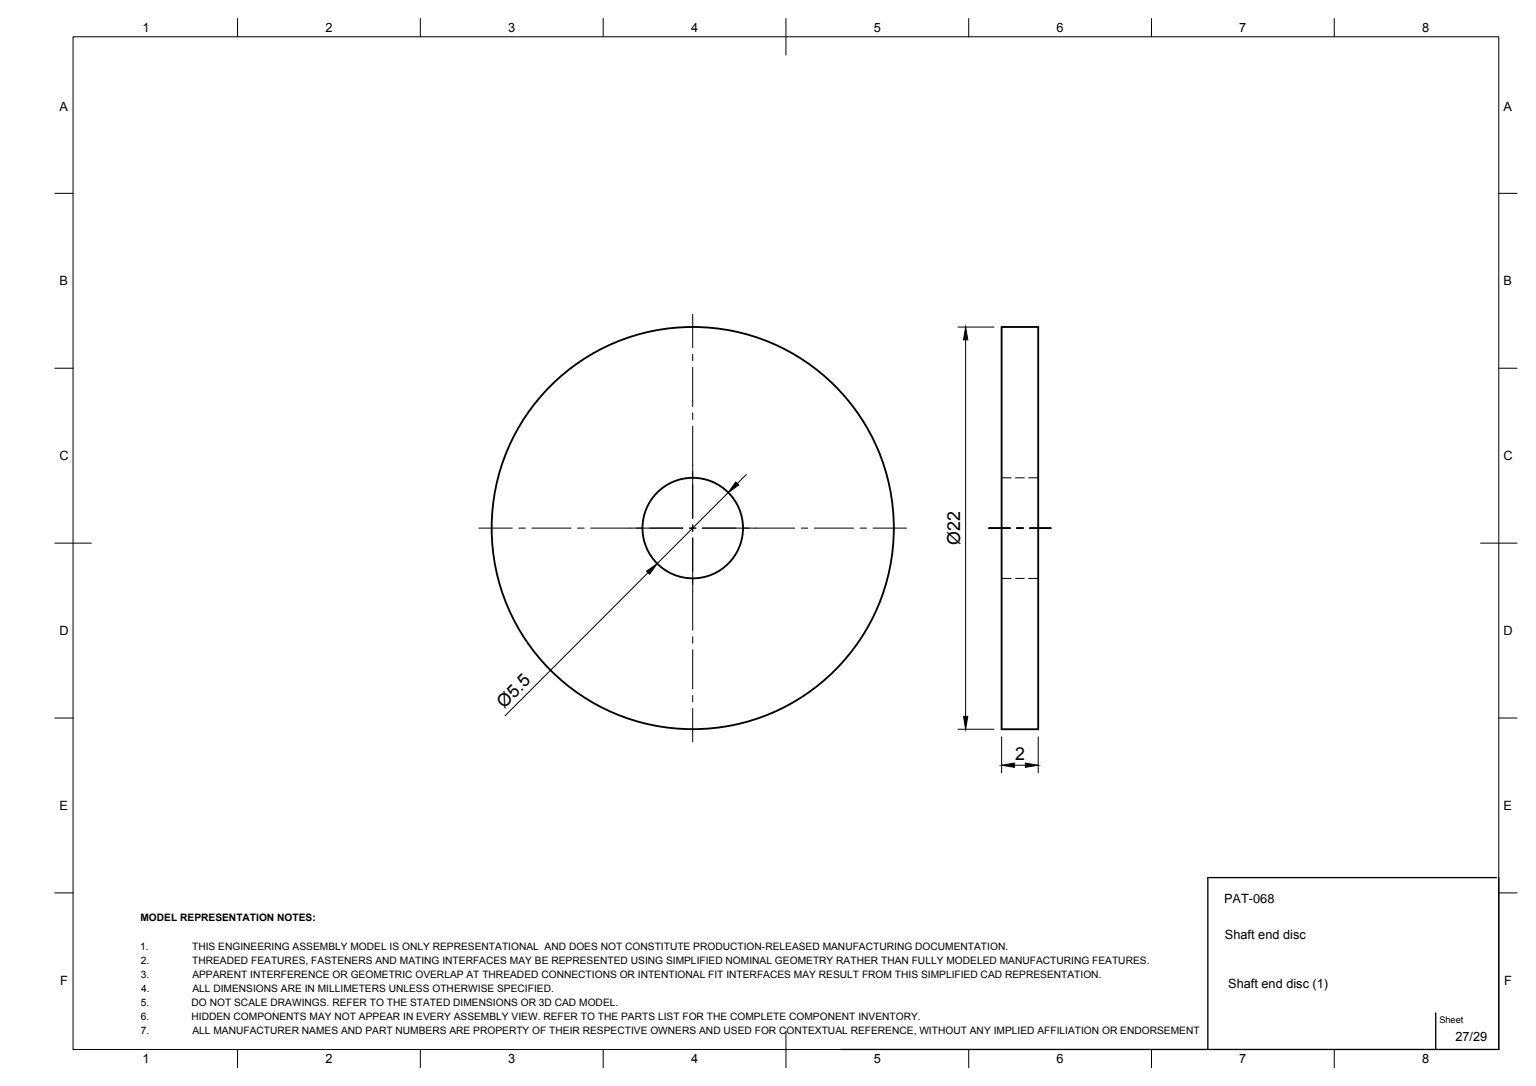
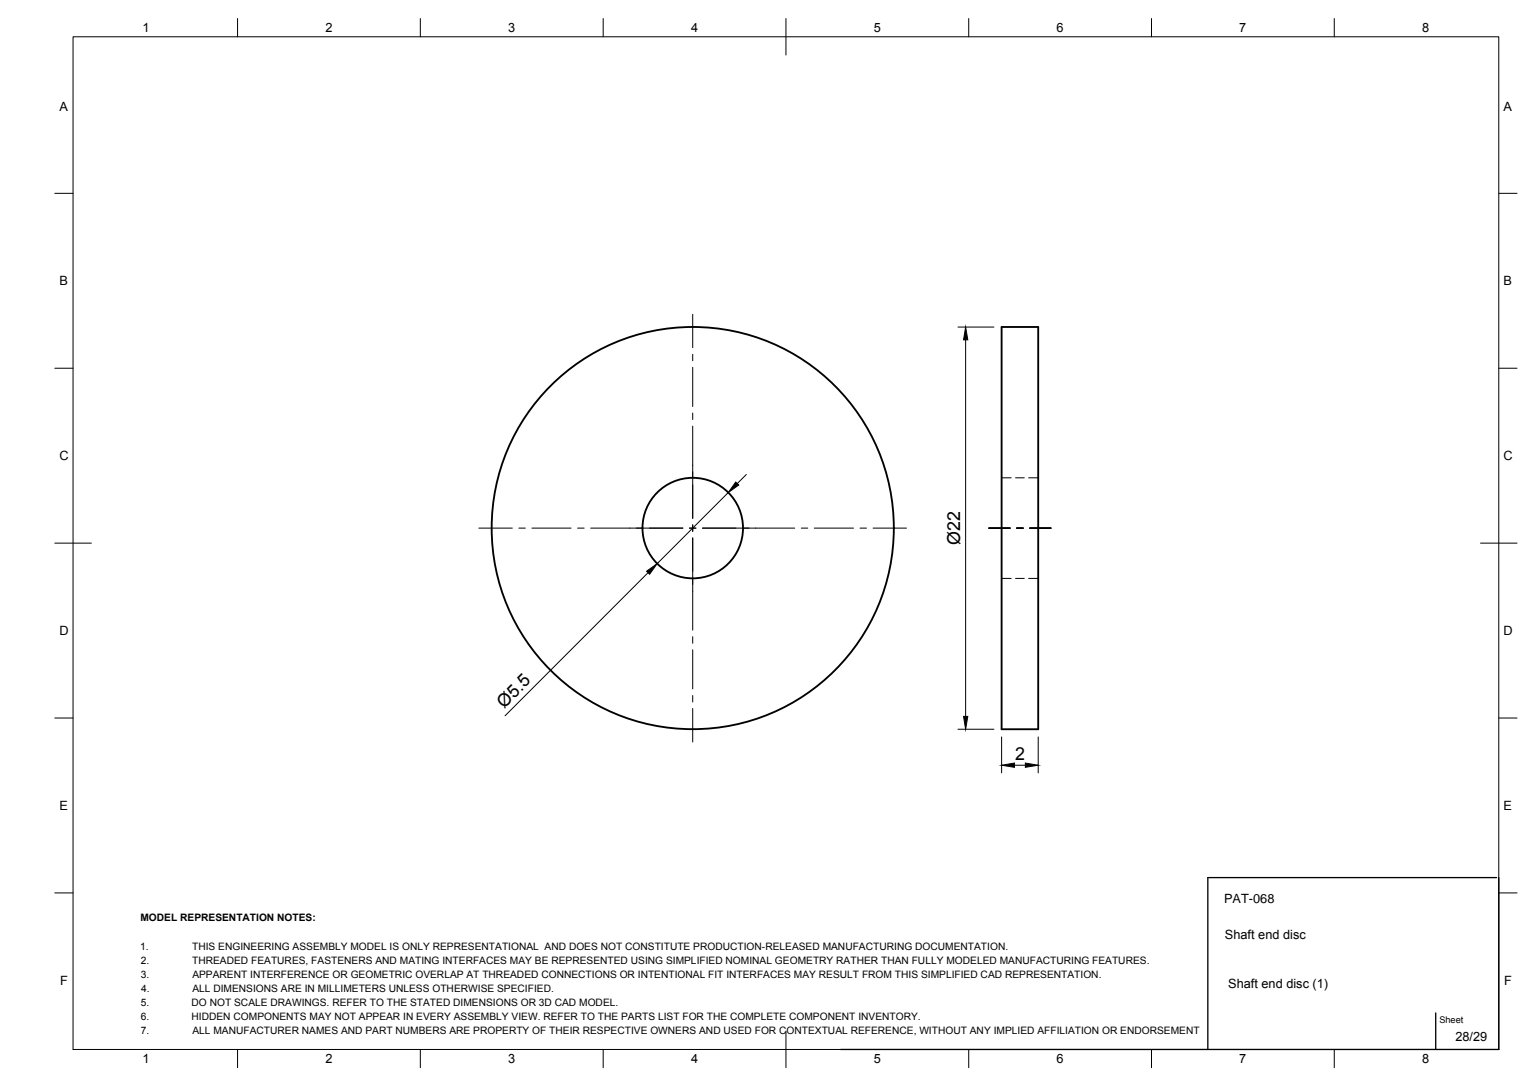
ISO-10303-21;
HEADER;
/* Generated by software containing ST-Developer
 * from STEP Tools, Inc. (www.steptools.com) 
 */

FILE_DESCRIPTION(
/* description */ ('Line shaft on three pillow blocks'),
/* implementation_level */ '2;1');

FILE_NAME(
/* name */ 'Shaft end disc.step',
/* time_stamp */ '2026-10-27T10:49:19-07:00',
/* author */ (''),
/* organization */ (''),
/* preprocessor_version */ 'ST-DEVELOPER v20.2',
/* originating_system */ 'Autodesk Translation Framework v15.17.0.0',
/* authorisation */ '');

FILE_SCHEMA (('AUTOMOTIVE_DESIGN { 1 0 10303 214 3 1 1 }'));
ENDSEC;

DATA;
#10=MECHANICAL_DESIGN_GEOMETRIC_PRESENTATION_REPRESENTATION('',(#361),#8377);
#306=SHAPE_REPRESENTATION_RELATIONSHIP('SRR','None',#8523,#333);
#333=ADVANCED_BREP_SHAPE_REPRESENTATION('',(#387),#8372);
#361=STYLED_ITEM('',(#8718),#387);
#387=MANIFOLD_SOLID_BREP('Body1',#4349);
#482=FACE_BOUND('',#1205,.T.);
#483=FACE_BOUND('',#1207,.T.);
#620=PLANE('',#5066);
#621=PLANE('',#5067);
#859=FACE_OUTER_BOUND('',#1202,.T.);
#860=FACE_OUTER_BOUND('',#1203,.T.);
#861=FACE_OUTER_BOUND('',#1204,.T.);
#862=FACE_OUTER_BOUND('',#1206,.T.);
#1202=EDGE_LOOP('',(#3815,#3816,#3817,#3818));
#1203=EDGE_LOOP('',(#3819,#3820,#3821,#3822));
#1204=EDGE_LOOP('',(#3823));
#1205=EDGE_LOOP('',(#3824));
#1206=EDGE_LOOP('',(#3825));
#1207=EDGE_LOOP('',(#3826));
#1509=LINE('',#8097,#1836);
#1510=LINE('',#8103,#1837);
#1836=VECTOR('',#6220,0.275);
#1837=VECTOR('',#6227,1.1);
#2048=CIRCLE('',#5061,0.275);
#2049=CIRCLE('',#5062,0.275);
#2050=CIRCLE('',#5064,1.1);
#2051=CIRCLE('',#5065,1.1);
#2363=VERTEX_POINT('',#8094);
#2364=VERTEX_POINT('',#8096);
#2365=VERTEX_POINT('',#8100);
#2366=VERTEX_POINT('',#8102);
#2856=EDGE_CURVE('',#2363,#2363,#2048,.T.);
#2857=EDGE_CURVE('',#2363,#2364,#1509,.T.);
#2858=EDGE_CURVE('',#2364,#2364,#2049,.T.);
#2859=EDGE_CURVE('',#2365,#2365,#2050,.T.);
#2860=EDGE_CURVE('',#2365,#2366,#1510,.T.);
#2861=EDGE_CURVE('',#2366,#2366,#2051,.T.);
#3815=ORIENTED_EDGE('',*,*,#2856,.F.);
#3816=ORIENTED_EDGE('',*,*,#2857,.T.);
#3817=ORIENTED_EDGE('',*,*,#2858,.T.);
#3818=ORIENTED_EDGE('',*,*,#2857,.F.);
#3819=ORIENTED_EDGE('',*,*,#2859,.F.);
#3820=ORIENTED_EDGE('',*,*,#2860,.T.);
#3821=ORIENTED_EDGE('',*,*,#2861,.T.);
#3822=ORIENTED_EDGE('',*,*,#2860,.F.);
#3823=ORIENTED_EDGE('',*,*,#2859,.T.);
#3824=ORIENTED_EDGE('',*,*,#2856,.T.);
#3825=ORIENTED_EDGE('',*,*,#2861,.F.);
#3826=ORIENTED_EDGE('',*,*,#2858,.F.);
#4065=CYLINDRICAL_SURFACE('',#5060,0.275);
#4066=CYLINDRICAL_SURFACE('',#5063,1.1);
#4277=ADVANCED_FACE('',(#859),#4065,.F.);
#4278=ADVANCED_FACE('',(#860),#4066,.T.);
#4279=ADVANCED_FACE('',(#861,#482),#620,.T.);
#4280=ADVANCED_FACE('',(#862,#483),#621,.F.);
#4349=CLOSED_SHELL('',(#4277,#4278,#4279,#4280));
#5059=AXIS2_PLACEMENT_3D('',#8092,#6214,#6215);
#5060=AXIS2_PLACEMENT_3D('',#8093,#6216,#6217);
#5061=AXIS2_PLACEMENT_3D('',#8095,#6218,#6219);
#5062=AXIS2_PLACEMENT_3D('',#8098,#6221,#6222);
#5063=AXIS2_PLACEMENT_3D('',#8099,#6223,#6224);
#5064=AXIS2_PLACEMENT_3D('',#8101,#6225,#6226);
#5065=AXIS2_PLACEMENT_3D('',#8104,#6228,#6229);
#5066=AXIS2_PLACEMENT_3D('',#8105,#6230,#6231);
#5067=AXIS2_PLACEMENT_3D('',#8106,#6232,#6233);
#6214=DIRECTION('axis',(0.,0.,1.));
#6215=DIRECTION('refdir',(1.,0.,0.));
#6216=DIRECTION('center_axis',(0.,1.,0.));
#6217=DIRECTION('ref_axis',(1.,0.,0.));
#6218=DIRECTION('center_axis',(0.,-1.,0.));
#6219=DIRECTION('ref_axis',(1.,0.,0.));
#6220=DIRECTION('',(0.,-1.,0.));
#6221=DIRECTION('center_axis',(0.,-1.,0.));
#6222=DIRECTION('ref_axis',(1.,0.,0.));
#6223=DIRECTION('center_axis',(0.,1.,0.));
#6224=DIRECTION('ref_axis',(1.,0.,0.));
#6225=DIRECTION('center_axis',(0.,1.,0.));
#6226=DIRECTION('ref_axis',(1.,0.,0.));
#6227=DIRECTION('',(0.,-1.,0.));
#6228=DIRECTION('center_axis',(0.,1.,0.));
#6229=DIRECTION('ref_axis',(1.,0.,0.));
#6230=DIRECTION('center_axis',(0.,1.,0.));
#6231=DIRECTION('ref_axis',(1.,0.,0.));
#6232=DIRECTION('center_axis',(0.,1.,0.));
#6233=DIRECTION('ref_axis',(1.,0.,0.));
#8092=CARTESIAN_POINT('',(0.,0.,0.));
#8093=CARTESIAN_POINT('Origin',(0.,-4.7,4.53));
#8094=CARTESIAN_POINT('',(-0.275,-4.5,4.53));
#8095=CARTESIAN_POINT('Origin',(0.,-4.5,4.53));
#8096=CARTESIAN_POINT('',(-0.275,-4.7,4.53));
#8097=CARTESIAN_POINT('',(-0.275,-4.7,4.53));
#8098=CARTESIAN_POINT('Origin',(0.,-4.7,4.53));
#8099=CARTESIAN_POINT('Origin',(0.,-4.7,4.53));
#8100=CARTESIAN_POINT('',(-1.1,-4.5,4.53));
#8101=CARTESIAN_POINT('Origin',(0.,-4.5,4.53));
#8102=CARTESIAN_POINT('',(-1.1,-4.7,4.53));
#8103=CARTESIAN_POINT('',(-1.1,-4.7,4.53));
#8104=CARTESIAN_POINT('Origin',(0.,-4.7,4.53));
#8105=CARTESIAN_POINT('Origin',(0.,-4.5,4.53));
#8106=CARTESIAN_POINT('Origin',(0.,-4.7,4.53));
#8340=UNCERTAINTY_MEASURE_WITH_UNIT(LENGTH_MEASURE(0.001),#8378,
'DISTANCE_ACCURACY_VALUE',
'Maximum model space distance between geometric entities at asserted c
onnectivities');
#8345=UNCERTAINTY_MEASURE_WITH_UNIT(LENGTH_MEASURE(0.001),#8378,
'DISTANCE_ACCURACY_VALUE',
'Maximum model space distance between geometric entities at asserted c
onnectivities');
#8372=(
GEOMETRIC_REPRESENTATION_CONTEXT(3)
GLOBAL_UNCERTAINTY_ASSIGNED_CONTEXT((#8340))
GLOBAL_UNIT_ASSIGNED_CONTEXT((#8378,#8380,#8381))
REPRESENTATION_CONTEXT('','3D')
);
#8377=(
GEOMETRIC_REPRESENTATION_CONTEXT(3)
GLOBAL_UNCERTAINTY_ASSIGNED_CONTEXT((#8345))
GLOBAL_UNIT_ASSIGNED_CONTEXT((#8378,#8380,#8381))
REPRESENTATION_CONTEXT('','3D')
);
#8378=(
LENGTH_UNIT()
NAMED_UNIT(*)
SI_UNIT(.CENTI.,.METRE.)
);
#8380=(
NAMED_UNIT(*)
PLANE_ANGLE_UNIT()
SI_UNIT($,.RADIAN.)
);
#8381=(
NAMED_UNIT(*)
SI_UNIT($,.STERADIAN.)
SOLID_ANGLE_UNIT()
);
#8408=SHAPE_DEFINITION_REPRESENTATION(#8475,#8523);
#8475=PRODUCT_DEFINITION_SHAPE('',$,#8555);
#8523=SHAPE_REPRESENTATION('',(#5059),#8372);
#8528=PRODUCT_DEFINITION_CONTEXT('part definition',#8623,'design');
#8555=PRODUCT_DEFINITION('Shaft end disc','Shaft end disc',#8586,#8528);
#8586=PRODUCT_DEFINITION_FORMATION('',$,#8651);
#8623=APPLICATION_CONTEXT(
'Core Data for Automotive Mechanical Design Process');
#8624=PRODUCT_CONTEXT('part definition',#8623,'mechanical');
#8651=PRODUCT('Shaft end disc','Shaft end disc','Shaft end disc',(#8624));
#8712=COLOUR_RGB('Grey',0.48,0.52,0.57);
#8713=FILL_AREA_STYLE_COLOUR('',#8712);
#8714=FILL_AREA_STYLE('',(#8713));
#8715=SURFACE_STYLE_FILL_AREA(#8714);
#8716=SURFACE_SIDE_STYLE('',(#8715));
#8717=SURFACE_STYLE_USAGE(.BOTH.,#8716);
#8718=PRESENTATION_STYLE_ASSIGNMENT((#8717));
ENDSEC;
END-ISO-10303-21;
